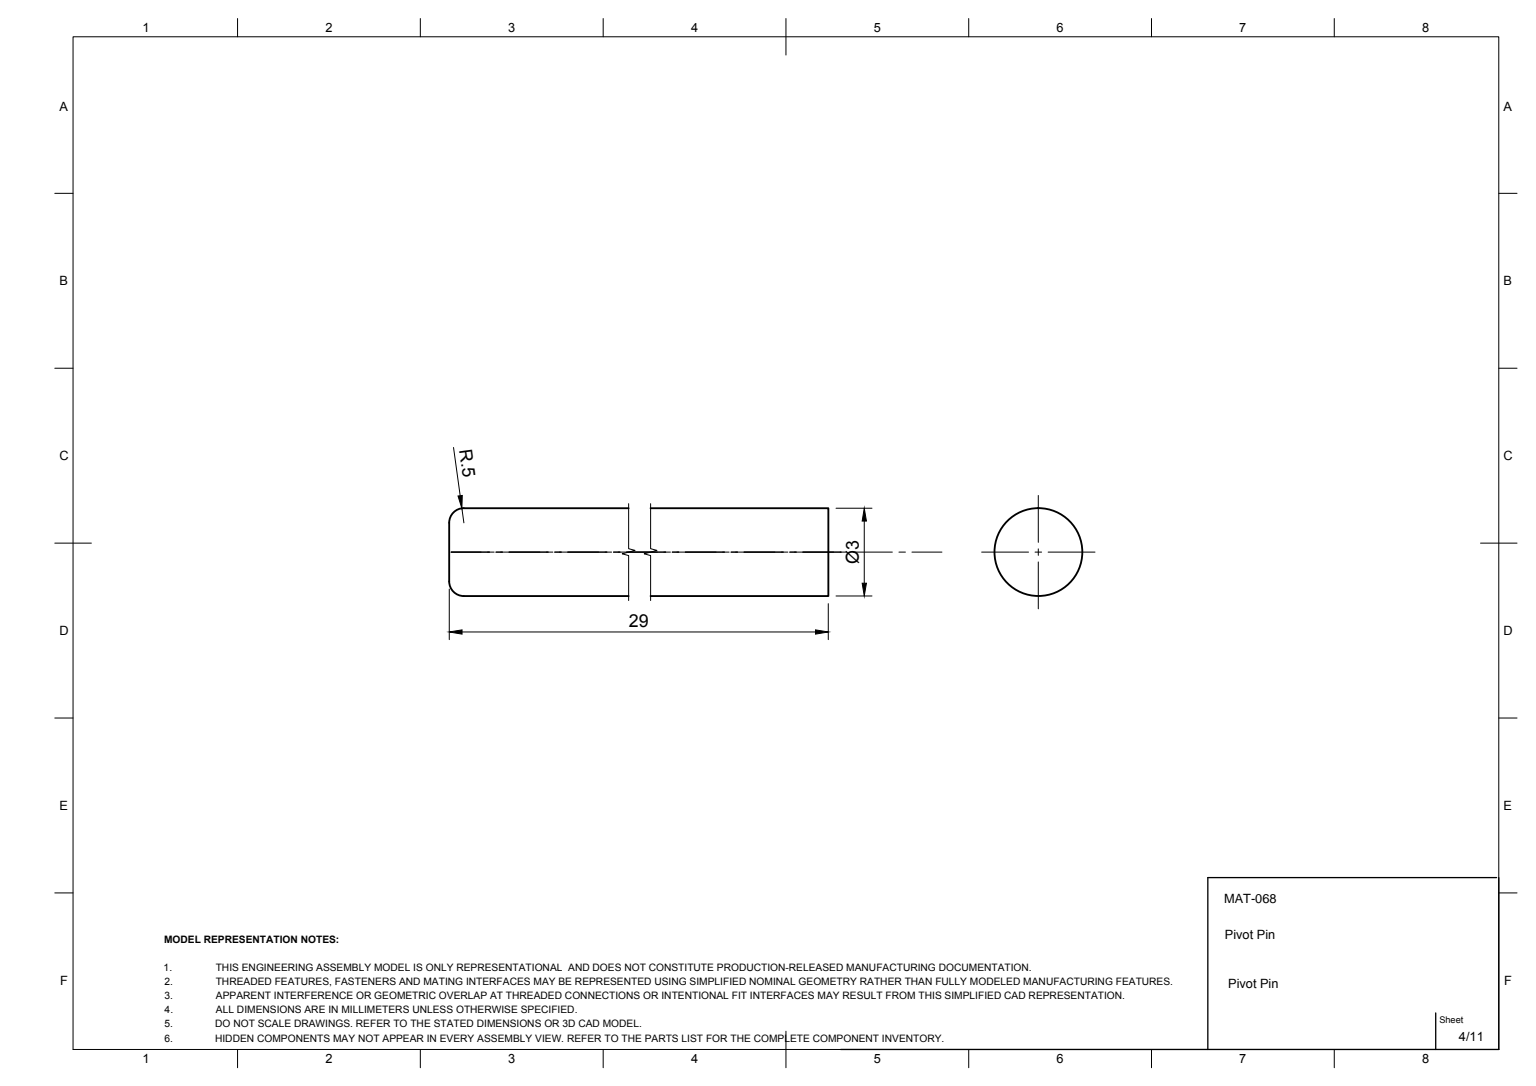
ISO-10303-21;
HEADER;
/* Generated by software containing ST-Developer
 * from STEP Tools, Inc. (www.steptools.com) 
 */

FILE_DESCRIPTION(
/* description */ ('CAx-IF Rec.Pracs.---Representation and Presentation of Product Manufa
cturing Information (PMI)---4.0---2014-10-13'),
/* implementation_level */ '2;1');

FILE_NAME(
/* name */ 'Pivot Pin.step',
/* time_stamp */ '2026-10-24T16:53:48-07:00',
/* author */ (''),
/* organization */ (''),
/* preprocessor_version */ 'ST-DEVELOPER v20.2',
/* originating_system */ 'Autodesk Translation Framework v15.17.0.0',
/* authorisation */ '');

FILE_SCHEMA (('AP242_MANAGED_MODEL_BASED_3D_ENGINEERING_MIM_LF { 1 0 10303 442 2 1 4 }'));
ENDSEC;

DATA;
#10=MECHANICAL_DESIGN_GEOMETRIC_PRESENTATION_REPRESENTATION('',(#3491),#107910);
#1136=TOROIDAL_SURFACE('',#45672,0.001,0.0005);
#3471=SHAPE_REPRESENTATION_RELATIONSHIP('SRR','None',#107949,#3481);
#3481=ADVANCED_BREP_SHAPE_REPRESENTATION('',(#3501),#107902);
#3491=STYLED_ITEM('',(#108008),#3501);
#3501=MANIFOLD_SOLID_BREP('Body1',#45539);
#3546=PLANE('',#45678);
#3547=PLANE('',#45679);
#3765=FACE_OUTER_BOUND('',#6691,.T.);
#3766=FACE_OUTER_BOUND('',#6692,.T.);
#3767=FACE_OUTER_BOUND('',#6693,.T.);
#3768=FACE_OUTER_BOUND('',#6694,.T.);
#6691=EDGE_LOOP('',(#28142,#28143,#28144,#28145));
#6692=EDGE_LOOP('',(#28146,#28147,#28148,#28149));
#6693=EDGE_LOOP('',(#28150));
#6694=EDGE_LOOP('',(#28151));
#9641=LINE('',#63374,#11625);
#11625=VECTOR('',#50416,0.0015);
#13611=CIRCLE('',#45673,0.00100000000001);
#13612=CIRCLE('',#45674,0.0005);
#13613=CIRCLE('',#45675,0.00150000000001);
#13614=CIRCLE('',#45677,0.00150000000001);
#17186=VERTEX_POINT('',#63367);
#17187=VERTEX_POINT('',#63369);
#17188=VERTEX_POINT('',#63373);
#21213=EDGE_CURVE('',#17186,#17186,#13611,.T.);
#21214=EDGE_CURVE('',#17186,#17187,#13612,.T.);
#21215=EDGE_CURVE('',#17187,#17187,#13613,.T.);
#21216=EDGE_CURVE('',#17187,#17188,#9641,.T.);
#21217=EDGE_CURVE('',#17188,#17188,#13614,.T.);
#28142=ORIENTED_EDGE('',*,*,#21213,.F.);
#28143=ORIENTED_EDGE('',*,*,#21214,.T.);
#28144=ORIENTED_EDGE('',*,*,#21215,.F.);
#28145=ORIENTED_EDGE('',*,*,#21214,.F.);
#28146=ORIENTED_EDGE('',*,*,#21215,.T.);
#28147=ORIENTED_EDGE('',*,*,#21216,.T.);
#28148=ORIENTED_EDGE('',*,*,#21217,.T.);
#28149=ORIENTED_EDGE('',*,*,#21216,.F.);
#28150=ORIENTED_EDGE('',*,*,#21217,.F.);
#28151=ORIENTED_EDGE('',*,*,#21213,.T.);
#41962=CYLINDRICAL_SURFACE('',#45676,0.0015);
#42620=ADVANCED_FACE('',(#3765),#1136,.T.);
#42621=ADVANCED_FACE('',(#3766),#41962,.T.);
#42622=ADVANCED_FACE('',(#3767),#3546,.F.);
#42623=ADVANCED_FACE('',(#3768),#3547,.T.);
#45539=CLOSED_SHELL('',(#42620,#42621,#42622,#42623));
#45671=AXIS2_PLACEMENT_3D('',#63365,#50404,#50405);
#45672=AXIS2_PLACEMENT_3D('',#63366,#50406,#50407);
#45673=AXIS2_PLACEMENT_3D('',#63368,#50408,#50409);
#45674=AXIS2_PLACEMENT_3D('',#63370,#50410,#50411);
#45675=AXIS2_PLACEMENT_3D('',#63371,#50412,#50413);
#45676=AXIS2_PLACEMENT_3D('',#63372,#50414,#50415);
#45677=AXIS2_PLACEMENT_3D('',#63375,#50417,#50418);
#45678=AXIS2_PLACEMENT_3D('',#63376,#50419,#50420);
#45679=AXIS2_PLACEMENT_3D('',#63377,#50421,#50422);
#50404=DIRECTION('axis',(0.,0.,1.));
#50405=DIRECTION('refdir',(1.,0.,0.));
#50406=DIRECTION('center_axis',(0.,0.,-1.));
#50407=DIRECTION('ref_axis',(-1.,0.,0.));
#50408=DIRECTION('center_axis',(0.,0.,-1.));
#50409=DIRECTION('ref_axis',(-1.,0.,0.));
#50410=DIRECTION('center_axis',(0.,-1.,0.));
#50411=DIRECTION('ref_axis',(1.,0.,0.));
#50412=DIRECTION('center_axis',(0.,0.,1.));
#50413=DIRECTION('ref_axis',(-1.,0.,0.));
#50414=DIRECTION('center_axis',(0.,0.,-1.));
#50415=DIRECTION('ref_axis',(-1.,0.,0.));
#50416=DIRECTION('',(0.,0.,1.));
#50417=DIRECTION('center_axis',(0.,0.,-1.));
#50418=DIRECTION('ref_axis',(-1.,0.,0.));
#50419=DIRECTION('center_axis',(0.,0.,-1.));
#50420=DIRECTION('ref_axis',(0.,-1.,0.));
#50421=DIRECTION('center_axis',(0.,0.,-1.));
#50422=DIRECTION('ref_axis',(0.,-1.,0.));
#63365=CARTESIAN_POINT('',(0.,0.,0.));
#63366=CARTESIAN_POINT('Origin',(-0.0186262178068916,-0.0128741814719618,
0.0571));
#63367=CARTESIAN_POINT('',(-0.0176262178068916,-0.0128741814719618,0.05660000000001));
#63368=CARTESIAN_POINT('Origin',(-0.0186262178069016,-0.0128741814719718,
0.05660000000001));
#63369=CARTESIAN_POINT('',(-0.0171262178068916,-0.0128741814719618,0.05710000000001));
#63370=CARTESIAN_POINT('Origin',(-0.0176262178068916,-0.0128741814719618,
0.0571));
#63371=CARTESIAN_POINT('Origin',(-0.0186262178069016,-0.0128741814719718,
0.05710000000001));
#63372=CARTESIAN_POINT('Origin',(-0.0186262178068916,-0.0128741814719618,
0.0856));
#63373=CARTESIAN_POINT('',(-0.0171262178068916,-0.0128741814719618,0.08560000000001));
#63374=CARTESIAN_POINT('',(-0.0171262178068916,-0.0128741814719618,0.0856));
#63375=CARTESIAN_POINT('Origin',(-0.0186262178069016,-0.0128741814719718,
0.08560000000001));
#63376=CARTESIAN_POINT('Origin',(-0.0186262178068916,-0.0128741814719618,
0.0856));
#63377=CARTESIAN_POINT('Origin',(-0.0186262178068916,-0.0128741814719618,
0.0566));
#107890=UNCERTAINTY_MEASURE_WITH_UNIT(LENGTH_MEASURE(1.E-5),#107911,
'DISTANCE_ACCURACY_VALUE',
'Maximum model space distance between geometric entities at asserted c
onnectivities');
#107898=UNCERTAINTY_MEASURE_WITH_UNIT(LENGTH_MEASURE(1.E-5),#107911,
'DISTANCE_ACCURACY_VALUE',
'Maximum model space distance between geometric entities at asserted c
onnectivities');
#107902=(
GEOMETRIC_REPRESENTATION_CONTEXT(3)
GLOBAL_UNCERTAINTY_ASSIGNED_CONTEXT((#107890))
GLOBAL_UNIT_ASSIGNED_CONTEXT((#107911,#107912,#107913))
REPRESENTATION_CONTEXT('','3D')
);
#107910=(
GEOMETRIC_REPRESENTATION_CONTEXT(3)
GLOBAL_UNCERTAINTY_ASSIGNED_CONTEXT((#107898))
GLOBAL_UNIT_ASSIGNED_CONTEXT((#107911,#107912,#107913))
REPRESENTATION_CONTEXT('','3D')
);
#107911=(
LENGTH_UNIT()
NAMED_UNIT(*)
SI_UNIT($,.METRE.)
);
#107912=(
NAMED_UNIT(*)
PLANE_ANGLE_UNIT()
SI_UNIT($,.RADIAN.)
);
#107913=(
NAMED_UNIT(*)
SI_UNIT($,.STERADIAN.)
SOLID_ANGLE_UNIT()
);
#107917=SHAPE_DEFINITION_REPRESENTATION(#107928,#107949);
#107928=PRODUCT_DEFINITION_SHAPE('',$,#107961);
#107949=SHAPE_REPRESENTATION('',(#45671),#107902);
#107957=PRODUCT_DEFINITION_CONTEXT('part definition',#107992,'design');
#107961=PRODUCT_DEFINITION('Pivot Pin','Pivot Pin',#107972,#107957);
#107972=PRODUCT_DEFINITION_FORMATION('',$,#107997);
#107992=APPLICATION_CONTEXT('Managed model based 3d engineering');
#107993=PRODUCT_CONTEXT('part definition',#107992,'mechanical');
#107997=PRODUCT('Pivot Pin','Pivot Pin',
'LEGAL AND USAGE DISCLAIMER: this Data/Model is provided \X2\201C\X0\A
S IS\X2\201D\X0\ for informational and representational only. It is a 
geometric approximation and is NOT engineered, certified, or guarantee
d for dimensional accuracy, exact tolerances, or production-level prec
ision. Vendor disclaims all implied warranties including fitness for a
 particular purpose. DO NOT USE FOR DIRECT PHYSICAL MANUFACTURING, AUT
OMATED PRODUCTION, OR SAFETY-CRITICAL SYSTEMS without independent engi
neering verification and resolution of any design discrepancies.',(#107993));
#108008=PRESENTATION_STYLE_ASSIGNMENT((#108015));
#108015=SURFACE_STYLE_USAGE(.BOTH.,#108022);
#108022=SURFACE_SIDE_STYLE('',(#108029));
#108029=SURFACE_STYLE_FILL_AREA(#108036);
#108036=FILL_AREA_STYLE('Opaque(246,246,243)',(#108043));
#108043=FILL_AREA_STYLE_COLOUR('Opaque(246,246,243)',#108050);
#108050=COLOUR_RGB('Opaque(246,246,243)',0.964705882352941,0.964705882352941,
0.952941176470588);
ENDSEC;
END-ISO-10303-21;
